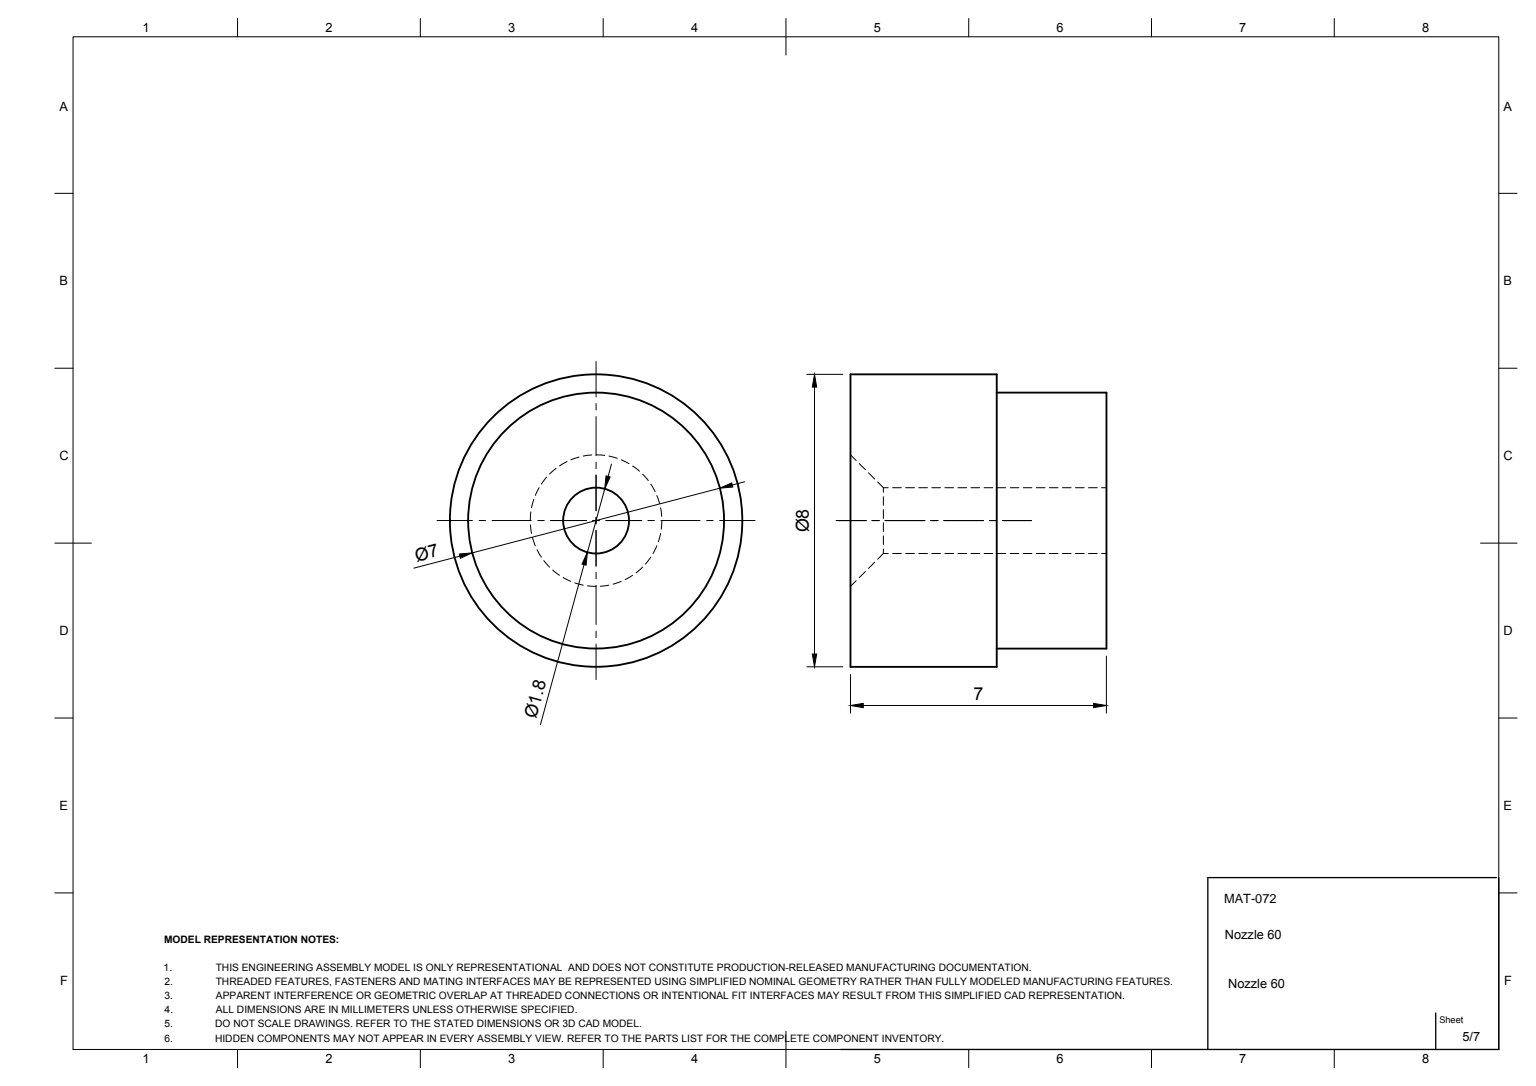
ISO-10303-21;
HEADER;
/* Generated by software containing ST-Developer
 * from STEP Tools, Inc. (www.steptools.com) 
 */

FILE_DESCRIPTION(
/* description */ (''),
/* implementation_level */ '2;1');

FILE_NAME(
/* name */ 'Nozzle 60.step',
/* time_stamp */ '2026-10-24T10:30:45-07:00',
/* author */ (''),
/* organization */ (''),
/* preprocessor_version */ 'ST-DEVELOPER v20.2',
/* originating_system */ 'Autodesk Translation Framework v15.15.0.0',
/* authorisation */ '');

FILE_SCHEMA (('AUTOMOTIVE_DESIGN { 1 0 10303 214 3 1 1 }'));
ENDSEC;

DATA;
#10=MECHANICAL_DESIGN_GEOMETRIC_PRESENTATION_REPRESENTATION('',(#79),#5183);
#64=CONICAL_SURFACE('',#2631,1.8,0.785398163397439);
#69=SHAPE_REPRESENTATION_RELATIONSHIP('SRR','None',#5216,#74);
#74=ADVANCED_BREP_SHAPE_REPRESENTATION('',(#84),#5180);
#79=STYLED_ITEM('',(#5247),#84);
#84=MANIFOLD_SOLID_BREP('Nozzle 60',#2365);
#135=FACE_BOUND('',#578,.T.);
#136=FACE_BOUND('',#580,.T.);
#137=FACE_BOUND('',#584,.T.);
#197=PLANE('',#2624);
#198=PLANE('',#2626);
#199=PLANE('',#2632);
#391=FACE_OUTER_BOUND('',#576,.T.);
#392=FACE_OUTER_BOUND('',#577,.T.);
#393=FACE_OUTER_BOUND('',#579,.T.);
#394=FACE_OUTER_BOUND('',#581,.T.);
#395=FACE_OUTER_BOUND('',#582,.T.);
#396=FACE_OUTER_BOUND('',#583,.T.);
#397=FACE_OUTER_BOUND('',#585,.T.);
#576=EDGE_LOOP('',(#2086,#2087,#2088,#2089));
#577=EDGE_LOOP('',(#2090));
#578=EDGE_LOOP('',(#2091));
#579=EDGE_LOOP('',(#2092));
#580=EDGE_LOOP('',(#2093));
#581=EDGE_LOOP('',(#2094,#2095,#2096,#2097));
#582=EDGE_LOOP('',(#2098,#2099,#2100,#2101));
#583=EDGE_LOOP('',(#2102));
#584=EDGE_LOOP('',(#2103));
#585=EDGE_LOOP('',(#2104,#2105,#2106,#2107));
#683=CIRCLE('',#2622,3.99999999999999);
#684=CIRCLE('',#2623,3.99999999999999);
#685=CIRCLE('',#2625,3.49999999999999);
#686=CIRCLE('',#2627,1.8);
#687=CIRCLE('',#2629,0.899999999999989);
#688=CIRCLE('',#2630,0.899999999999988);
#689=CIRCLE('',#2633,3.49999999999999);
#842=LINE('',#5084,#992);
#843=LINE('',#5096,#993);
#844=LINE('',#5099,#994);
#845=LINE('',#5104,#995);
#992=VECTOR('',#3214,3.99999999999999);
#993=VECTOR('',#3229,0.899999999999994);
#994=VECTOR('',#3234,1.8);
#995=VECTOR('',#3241,3.49999999999999);
#1189=VERTEX_POINT('',#5081);
#1190=VERTEX_POINT('',#5083);
#1191=VERTEX_POINT('',#5087);
#1192=VERTEX_POINT('',#5090);
#1193=VERTEX_POINT('',#5093);
#1194=VERTEX_POINT('',#5095);
#1195=VERTEX_POINT('',#5101);
#1491=EDGE_CURVE('',#1189,#1189,#683,.T.);
#1492=EDGE_CURVE('',#1189,#1190,#842,.T.);
#1493=EDGE_CURVE('',#1190,#1190,#684,.T.);
#1494=EDGE_CURVE('',#1191,#1191,#685,.T.);
#1495=EDGE_CURVE('',#1192,#1192,#686,.T.);
#1496=EDGE_CURVE('',#1193,#1193,#687,.T.);
#1497=EDGE_CURVE('',#1193,#1194,#843,.T.);
#1498=EDGE_CURVE('',#1194,#1194,#688,.T.);
#1499=EDGE_CURVE('',#1194,#1192,#844,.T.);
#1500=EDGE_CURVE('',#1195,#1195,#689,.T.);
#1501=EDGE_CURVE('',#1191,#1195,#845,.T.);
#2086=ORIENTED_EDGE('',*,*,#1491,.T.);
#2087=ORIENTED_EDGE('',*,*,#1492,.T.);
#2088=ORIENTED_EDGE('',*,*,#1493,.F.);
#2089=ORIENTED_EDGE('',*,*,#1492,.F.);
#2090=ORIENTED_EDGE('',*,*,#1493,.T.);
#2091=ORIENTED_EDGE('',*,*,#1494,.F.);
#2092=ORIENTED_EDGE('',*,*,#1491,.F.);
#2093=ORIENTED_EDGE('',*,*,#1495,.F.);
#2094=ORIENTED_EDGE('',*,*,#1496,.T.);
#2095=ORIENTED_EDGE('',*,*,#1497,.T.);
#2096=ORIENTED_EDGE('',*,*,#1498,.T.);
#2097=ORIENTED_EDGE('',*,*,#1497,.F.);
#2098=ORIENTED_EDGE('',*,*,#1498,.F.);
#2099=ORIENTED_EDGE('',*,*,#1499,.T.);
#2100=ORIENTED_EDGE('',*,*,#1495,.T.);
#2101=ORIENTED_EDGE('',*,*,#1499,.F.);
#2102=ORIENTED_EDGE('',*,*,#1500,.T.);
#2103=ORIENTED_EDGE('',*,*,#1496,.F.);
#2104=ORIENTED_EDGE('',*,*,#1494,.T.);
#2105=ORIENTED_EDGE('',*,*,#1501,.T.);
#2106=ORIENTED_EDGE('',*,*,#1500,.F.);
#2107=ORIENTED_EDGE('',*,*,#1501,.F.);
#2214=CYLINDRICAL_SURFACE('',#2621,3.99999999999999);
#2215=CYLINDRICAL_SURFACE('',#2628,0.899999999999993);
#2216=CYLINDRICAL_SURFACE('',#2634,3.49999999999999);
#2342=ADVANCED_FACE('',(#391),#2214,.T.);
#2343=ADVANCED_FACE('',(#392,#135),#197,.T.);
#2344=ADVANCED_FACE('',(#393,#136),#198,.F.);
#2345=ADVANCED_FACE('',(#394),#2215,.F.);
#2346=ADVANCED_FACE('',(#395),#64,.F.);
#2347=ADVANCED_FACE('',(#396,#137),#199,.T.);
#2348=ADVANCED_FACE('',(#397),#2216,.T.);
#2365=CLOSED_SHELL('',(#2342,#2343,#2344,#2345,#2346,#2347,#2348));
#2620=AXIS2_PLACEMENT_3D('',#5079,#3208,#3209);
#2621=AXIS2_PLACEMENT_3D('',#5080,#3210,#3211);
#2622=AXIS2_PLACEMENT_3D('',#5082,#3212,#3213);
#2623=AXIS2_PLACEMENT_3D('',#5085,#3215,#3216);
#2624=AXIS2_PLACEMENT_3D('',#5086,#3217,#3218);
#2625=AXIS2_PLACEMENT_3D('',#5088,#3219,#3220);
#2626=AXIS2_PLACEMENT_3D('',#5089,#3221,#3222);
#2627=AXIS2_PLACEMENT_3D('',#5091,#3223,#3224);
#2628=AXIS2_PLACEMENT_3D('',#5092,#3225,#3226);
#2629=AXIS2_PLACEMENT_3D('',#5094,#3227,#3228);
#2630=AXIS2_PLACEMENT_3D('',#5097,#3230,#3231);
#2631=AXIS2_PLACEMENT_3D('',#5098,#3232,#3233);
#2632=AXIS2_PLACEMENT_3D('',#5100,#3235,#3236);
#2633=AXIS2_PLACEMENT_3D('',#5102,#3237,#3238);
#2634=AXIS2_PLACEMENT_3D('',#5103,#3239,#3240);
#3208=DIRECTION('axis',(0.,0.,1.));
#3209=DIRECTION('refdir',(1.,0.,0.));
#3210=DIRECTION('center_axis',(-0.433012701892223,0.866025403784436,-0.250000000000002));
#3211=DIRECTION('ref_axis',(-0.894427190999914,-0.447213595499962,0.));
#3212=DIRECTION('center_axis',(0.433012701892223,-0.866025403784436,0.250000000000002));
#3213=DIRECTION('ref_axis',(0.894427190999914,0.447213595499962,0.));
#3214=DIRECTION('',(0.433012701892223,-0.866025403784436,0.250000000000002));
#3215=DIRECTION('center_axis',(0.433012701892223,-0.866025403784436,0.250000000000002));
#3216=DIRECTION('ref_axis',(0.894427190999914,0.447213595499962,0.));
#3217=DIRECTION('center_axis',(0.433012701892223,-0.866025403784436,0.250000000000002));
#3218=DIRECTION('ref_axis',(0.5,0.,-0.866025403784439));
#3219=DIRECTION('center_axis',(0.433012701892223,-0.866025403784437,0.250000000000002));
#3220=DIRECTION('ref_axis',(0.894427190999914,0.447213595499962,0.));
#3221=DIRECTION('center_axis',(0.433012701892223,-0.866025403784436,0.250000000000002));
#3222=DIRECTION('ref_axis',(0.5,0.,-0.866025403784439));
#3223=DIRECTION('center_axis',(-0.433012701892223,0.866025403784436,-0.250000000000002));
#3224=DIRECTION('ref_axis',(-0.894427190999914,-0.447213595499962,0.));
#3225=DIRECTION('center_axis',(-0.433012701892223,0.866025403784436,-0.250000000000002));
#3226=DIRECTION('ref_axis',(-0.894427190999914,-0.447213595499962,0.));
#3227=DIRECTION('center_axis',(0.433012701892223,-0.866025403784437,0.250000000000002));
#3228=DIRECTION('ref_axis',(0.894427190999914,0.447213595499962,0.));
#3229=DIRECTION('',(-0.433012701892223,0.866025403784436,-0.250000000000002));
#3230=DIRECTION('center_axis',(-0.433012701892223,0.866025403784436,-0.250000000000002));
#3231=DIRECTION('ref_axis',(-0.894427190999914,-0.447213595499962,0.));
#3232=DIRECTION('center_axis',(-0.433012701892223,0.866025403784436,-0.250000000000002));
#3233=DIRECTION('ref_axis',(-0.894427190999914,-0.447213595499962,0.));
#3234=DIRECTION('',(0.326269314185767,0.928600201712636,-0.17677669529664));
#3235=DIRECTION('center_axis',(0.433012701892223,-0.866025403784437,0.250000000000002));
#3236=DIRECTION('ref_axis',(0.5,0.,-0.866025403784439));
#3237=DIRECTION('center_axis',(0.433012701892223,-0.866025403784437,0.250000000000002));
#3238=DIRECTION('ref_axis',(0.894427190999914,0.447213595499962,0.));
#3239=DIRECTION('center_axis',(-0.433012701892223,0.866025403784436,-0.250000000000002));
#3240=DIRECTION('ref_axis',(-0.894427190999914,-0.447213595499962,0.));
#3241=DIRECTION('',(0.433012701892223,-0.866025403784436,0.250000000000002));
#5079=CARTESIAN_POINT('',(0.,0.,0.));
#5080=CARTESIAN_POINT('Origin',(-102.211351574804,130.535898384862,-71.0117513459462));
#5081=CARTESIAN_POINT('',(-100.365693618373,135.788854382,-72.0117513459462));
#5082=CARTESIAN_POINT('Origin',(-103.943402382373,134.,-72.0117513459462));
#5083=CARTESIAN_POINT('',(-98.6336428108046,132.324752766862,-71.0117513459462));
#5084=CARTESIAN_POINT('',(-98.6336428108046,132.324752766862,-71.0117513459462));
#5085=CARTESIAN_POINT('Origin',(-102.211351574804,130.535898384862,-71.0117513459462));
#5086=CARTESIAN_POINT('Origin',(-102.211351574804,130.535898384862,-71.0117513459462));
#5087=CARTESIAN_POINT('',(-99.0808564063046,132.101145969112,-71.0117513459462));
#5088=CARTESIAN_POINT('Origin',(-102.211351574804,130.535898384862,-71.0117513459462));
#5089=CARTESIAN_POINT('Origin',(-103.943402382373,134.,-72.0117513459462));
#5090=CARTESIAN_POINT('',(-102.333433438573,134.8049844719,-72.0117513459462));
#5091=CARTESIAN_POINT('Origin',(-103.943402382373,134.,-72.0117513459462));
#5092=CARTESIAN_POINT('Origin',(-103.943402382373,134.,-72.0117513459462));
#5093=CARTESIAN_POINT('',(-100.107328997228,128.340314409459,-70.2617513459462));
#5094=CARTESIAN_POINT('Origin',(-100.912313469128,127.937822173509,-70.2617513459462));
#5095=CARTESIAN_POINT('',(-102.74870647877,133.623069372544,-71.7867513459462));
#5096=CARTESIAN_POINT('',(-103.138417910473,134.40249223595,-72.0117513459462));
#5097=CARTESIAN_POINT('Origin',(-103.55369095067,133.220577136594,-71.7867513459462));
#5098=CARTESIAN_POINT('Origin',(-103.943402382373,134.,-72.0117513459462));
#5099=CARTESIAN_POINT('',(-102.333433438573,134.8049844719,-72.0117513459462));
#5100=CARTESIAN_POINT('Origin',(-100.912313469128,127.937822173509,-70.2617513459462));
#5101=CARTESIAN_POINT('',(-97.7818183006279,129.503069757759,-70.2617513459462));
#5102=CARTESIAN_POINT('Origin',(-100.912313469128,127.937822173509,-70.2617513459462));
#5103=CARTESIAN_POINT('Origin',(-100.912313469128,127.937822173509,-70.2617513459462));
#5104=CARTESIAN_POINT('',(-97.7818183006279,129.503069757759,-70.2617513459462));
#5173=UNCERTAINTY_MEASURE_WITH_UNIT(LENGTH_MEASURE(0.01),#5184,
'DISTANCE_ACCURACY_VALUE',
'Maximum model space distance between geometric entities at asserted c
onnectivities');
#5176=UNCERTAINTY_MEASURE_WITH_UNIT(LENGTH_MEASURE(0.01),#5184,
'DISTANCE_ACCURACY_VALUE',
'Maximum model space distance between geometric entities at asserted c
onnectivities');
#5180=(
GEOMETRIC_REPRESENTATION_CONTEXT(3)
GLOBAL_UNCERTAINTY_ASSIGNED_CONTEXT((#5173))
GLOBAL_UNIT_ASSIGNED_CONTEXT((#5184,#5186,#5187))
REPRESENTATION_CONTEXT('','3D')
);
#5183=(
GEOMETRIC_REPRESENTATION_CONTEXT(3)
GLOBAL_UNCERTAINTY_ASSIGNED_CONTEXT((#5176))
GLOBAL_UNIT_ASSIGNED_CONTEXT((#5184,#5186,#5187))
REPRESENTATION_CONTEXT('','3D')
);
#5184=(
LENGTH_UNIT()
NAMED_UNIT(*)
SI_UNIT(.MILLI.,.METRE.)
);
#5186=(
NAMED_UNIT(*)
PLANE_ANGLE_UNIT()
SI_UNIT($,.RADIAN.)
);
#5187=(
NAMED_UNIT(*)
SI_UNIT($,.STERADIAN.)
SOLID_ANGLE_UNIT()
);
#5191=SHAPE_DEFINITION_REPRESENTATION(#5197,#5216);
#5197=PRODUCT_DEFINITION_SHAPE('',$,#5223);
#5216=SHAPE_REPRESENTATION('',(#2620),#5180);
#5219=PRODUCT_DEFINITION_CONTEXT('part definition',#5239,'design');
#5223=PRODUCT_DEFINITION('Nozzle 60','Nozzle 60',#5229,#5219);
#5229=PRODUCT_DEFINITION_FORMATION('',$,#5244);
#5239=APPLICATION_CONTEXT(
'Core Data for Automotive Mechanical Design Process');
#5240=PRODUCT_CONTEXT('part definition',#5239,'mechanical');
#5244=PRODUCT('Nozzle 60','Nozzle 60',$,(#5240));
#5247=PRESENTATION_STYLE_ASSIGNMENT((#5248));
#5248=SURFACE_STYLE_USAGE(.BOTH.,#5249);
#5249=SURFACE_SIDE_STYLE('',(#5250));
#5250=SURFACE_STYLE_FILL_AREA(#5251);
#5251=FILL_AREA_STYLE('Steel - Satin',(#5252));
#5252=FILL_AREA_STYLE_COLOUR('Steel - Satin',#5253);
#5253=COLOUR_RGB('Steel - Satin',0.627450980392157,0.627450980392157,0.627450980392157);
ENDSEC;
END-ISO-10303-21;
